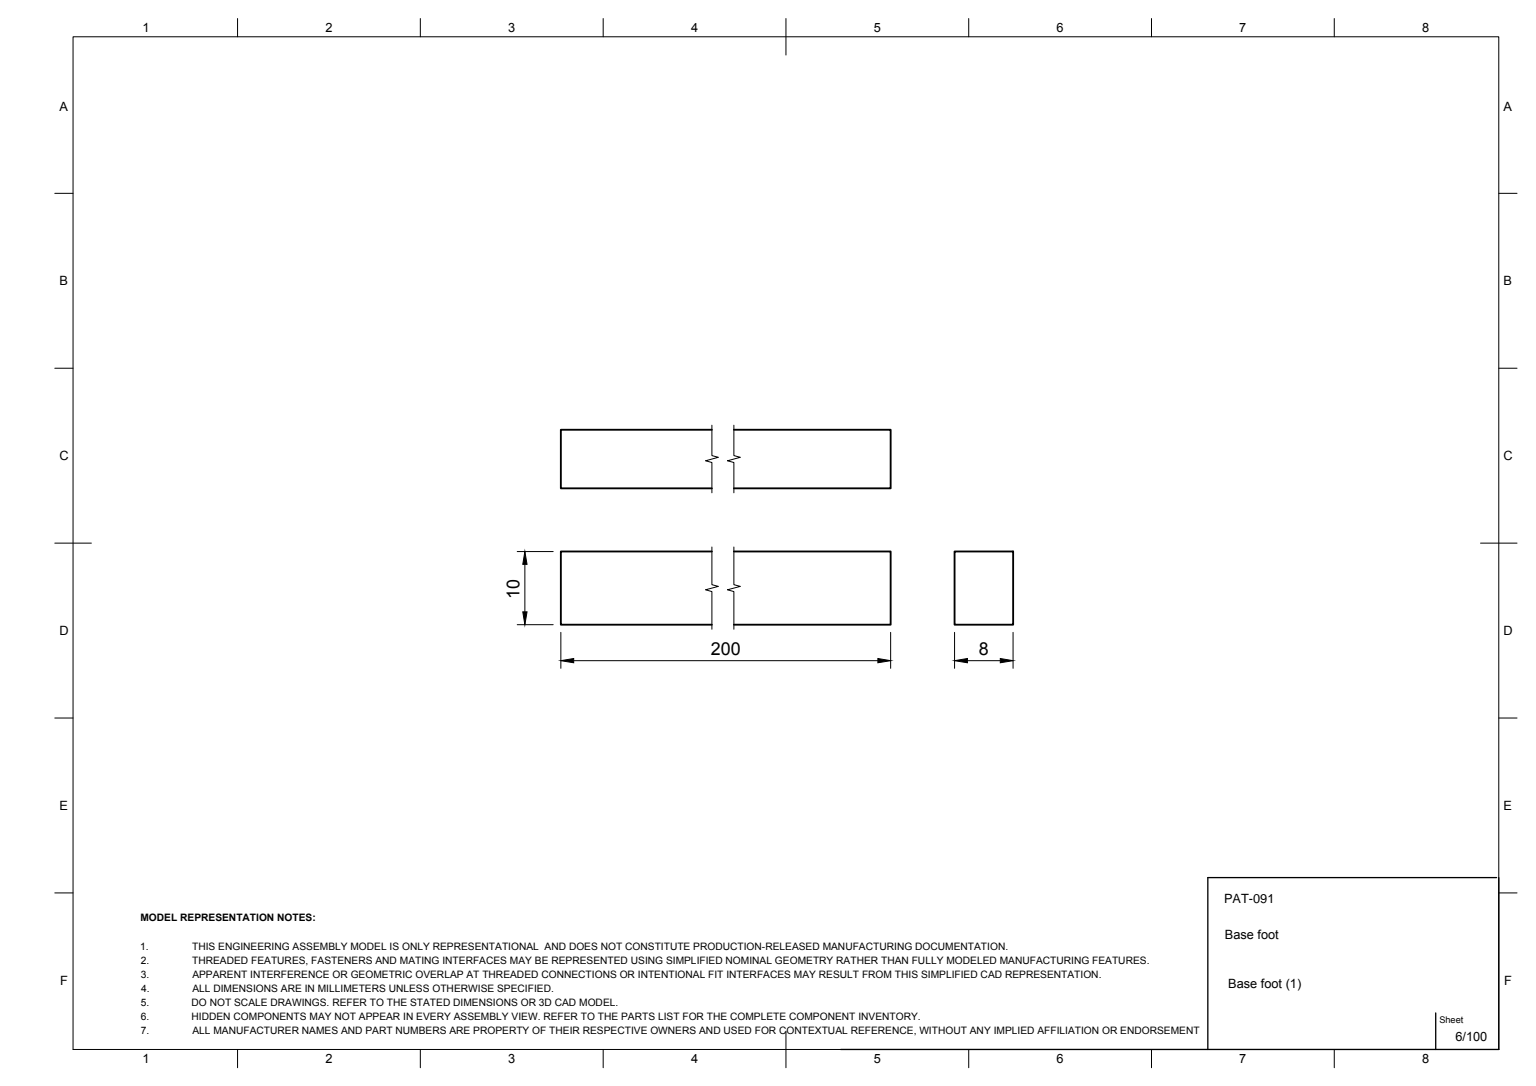
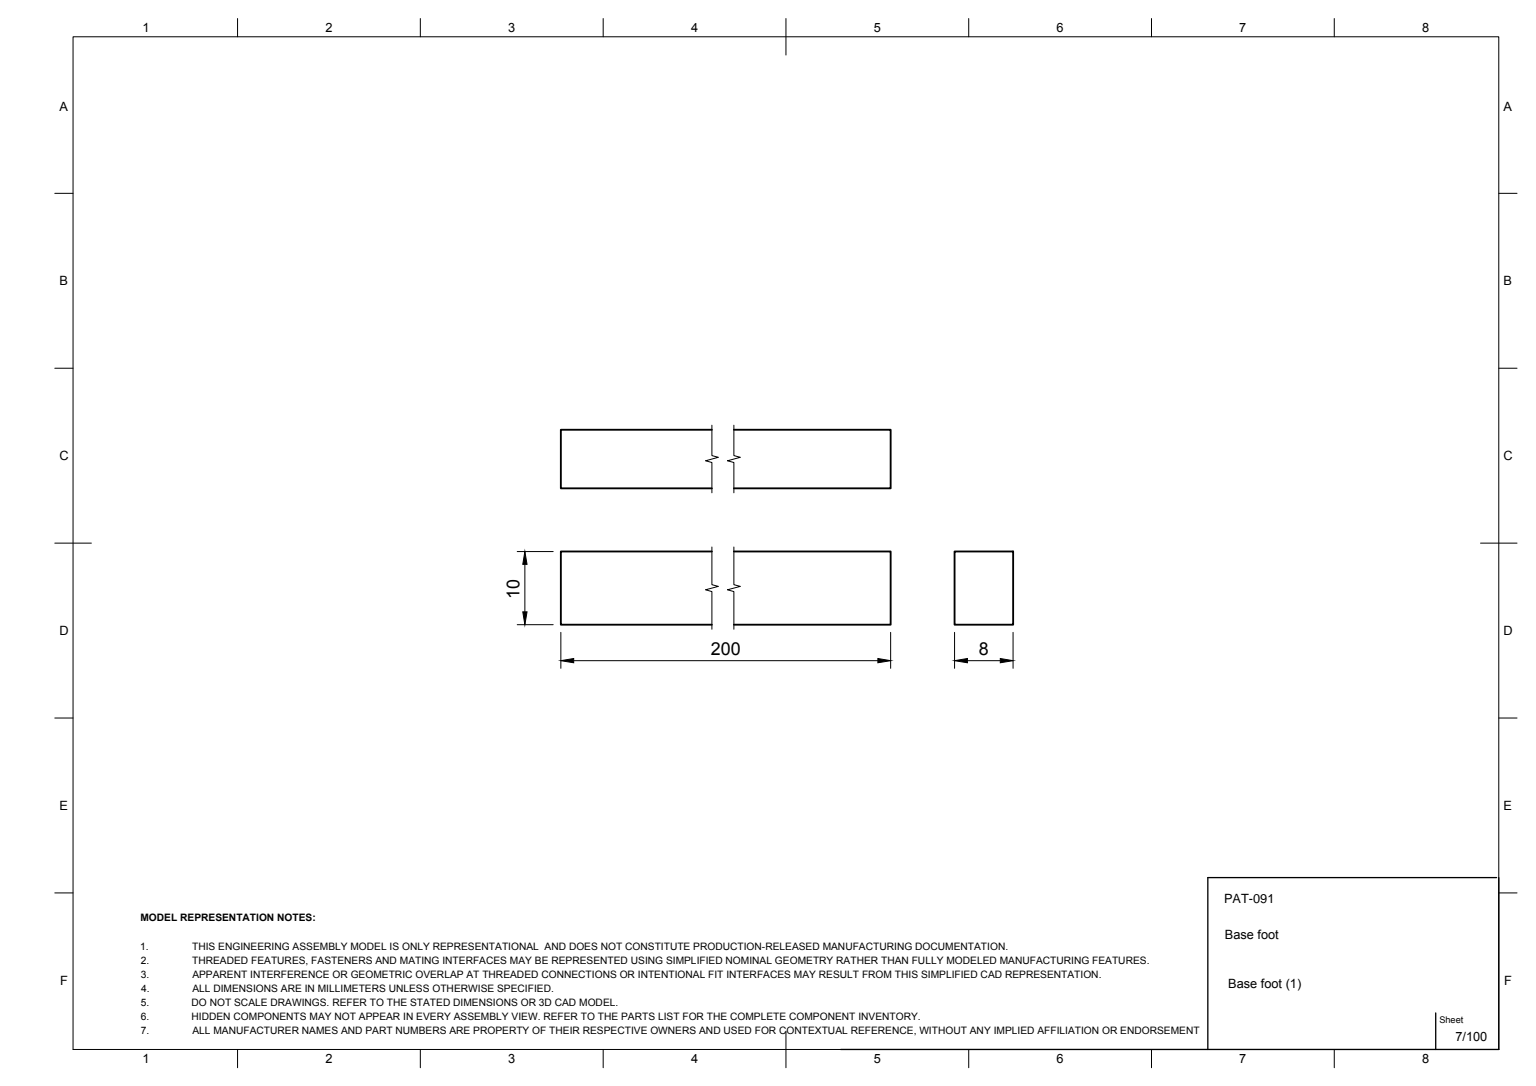
ISO-10303-21;
HEADER;
/* Generated by software containing ST-Developer
 * from STEP Tools, Inc. (www.steptools.com) 
 */

FILE_DESCRIPTION(
/* description */ ('PAT-091'),
/* implementation_level */ '2;1');

FILE_NAME(
/* name */ 'Base foot (1).step',
/* time_stamp */ '2026-10-27T15:34:44-07:00',
/* author */ (''),
/* organization */ (''),
/* preprocessor_version */ 'ST-DEVELOPER v20.2',
/* originating_system */ 'Autodesk Translation Framework v15.17.0.0',
/* authorisation */ '');

FILE_SCHEMA (('AUTOMOTIVE_DESIGN { 1 0 10303 214 3 1 1 }'));
ENDSEC;

DATA;
#10=MECHANICAL_DESIGN_GEOMETRIC_PRESENTATION_REPRESENTATION('',(#973),#25100);
#753=SHAPE_REPRESENTATION_RELATIONSHIP('SRR','None',#25514,#863);
#863=ADVANCED_BREP_SHAPE_REPRESENTATION('',(#1097),#24984);
#973=STYLED_ITEM('',(#26170),#1097);
#1097=MANIFOLD_SOLID_BREP('Body1',#13250);
#1652=PLANE('',#14626);
#1653=PLANE('',#14627);
#1654=PLANE('',#14628);
#1655=PLANE('',#14629);
#1656=PLANE('',#14630);
#1657=PLANE('',#14631);
#2083=FACE_OUTER_BOUND('',#2917,.T.);
#2084=FACE_OUTER_BOUND('',#2918,.T.);
#2085=FACE_OUTER_BOUND('',#2919,.T.);
#2086=FACE_OUTER_BOUND('',#2920,.T.);
#2087=FACE_OUTER_BOUND('',#2921,.T.);
#2088=FACE_OUTER_BOUND('',#2922,.T.);
#2917=EDGE_LOOP('',(#9068,#9069,#9070,#9071));
#2918=EDGE_LOOP('',(#9072,#9073,#9074,#9075));
#2919=EDGE_LOOP('',(#9076,#9077,#9078,#9079));
#2920=EDGE_LOOP('',(#9080,#9081,#9082,#9083));
#2921=EDGE_LOOP('',(#9084,#9085,#9086,#9087));
#2922=EDGE_LOOP('',(#9088,#9089,#9090,#9091));
#4156=LINE('',#21082,#4896);
#4157=LINE('',#21084,#4897);
#4158=LINE('',#21086,#4898);
#4159=LINE('',#21087,#4899);
#4160=LINE('',#21090,#4900);
#4161=LINE('',#21092,#4901);
#4162=LINE('',#21093,#4902);
#4163=LINE('',#21096,#4903);
#4164=LINE('',#21098,#4904);
#4165=LINE('',#21099,#4905);
#4166=LINE('',#21101,#4906);
#4167=LINE('',#21102,#4907);
#4896=VECTOR('',#16584,1.);
#4897=VECTOR('',#16585,1.);
#4898=VECTOR('',#16586,1.);
#4899=VECTOR('',#16587,1.);
#4900=VECTOR('',#16590,1.);
#4901=VECTOR('',#16591,1.);
#4902=VECTOR('',#16592,1.);
#4903=VECTOR('',#16595,1.);
#4904=VECTOR('',#16596,1.);
#4905=VECTOR('',#16597,1.);
#4906=VECTOR('',#16600,1.);
#4907=VECTOR('',#16601,1.);
#6415=VERTEX_POINT('',#21080);
#6416=VERTEX_POINT('',#21081);
#6417=VERTEX_POINT('',#21083);
#6418=VERTEX_POINT('',#21085);
#6419=VERTEX_POINT('',#21089);
#6420=VERTEX_POINT('',#21091);
#6421=VERTEX_POINT('',#21095);
#6422=VERTEX_POINT('',#21097);
#7469=EDGE_CURVE('',#6415,#6416,#4156,.T.);
#7470=EDGE_CURVE('',#6416,#6417,#4157,.T.);
#7471=EDGE_CURVE('',#6418,#6417,#4158,.T.);
#7472=EDGE_CURVE('',#6415,#6418,#4159,.T.);
#7473=EDGE_CURVE('',#6419,#6415,#4160,.T.);
#7474=EDGE_CURVE('',#6420,#6418,#4161,.T.);
#7475=EDGE_CURVE('',#6419,#6420,#4162,.T.);
#7476=EDGE_CURVE('',#6421,#6419,#4163,.T.);
#7477=EDGE_CURVE('',#6422,#6420,#4164,.T.);
#7478=EDGE_CURVE('',#6421,#6422,#4165,.T.);
#7479=EDGE_CURVE('',#6416,#6421,#4166,.T.);
#7480=EDGE_CURVE('',#6417,#6422,#4167,.T.);
#9068=ORIENTED_EDGE('',*,*,#7469,.T.);
#9069=ORIENTED_EDGE('',*,*,#7470,.T.);
#9070=ORIENTED_EDGE('',*,*,#7471,.F.);
#9071=ORIENTED_EDGE('',*,*,#7472,.F.);
#9072=ORIENTED_EDGE('',*,*,#7473,.T.);
#9073=ORIENTED_EDGE('',*,*,#7472,.T.);
#9074=ORIENTED_EDGE('',*,*,#7474,.F.);
#9075=ORIENTED_EDGE('',*,*,#7475,.F.);
#9076=ORIENTED_EDGE('',*,*,#7476,.T.);
#9077=ORIENTED_EDGE('',*,*,#7475,.T.);
#9078=ORIENTED_EDGE('',*,*,#7477,.F.);
#9079=ORIENTED_EDGE('',*,*,#7478,.F.);
#9080=ORIENTED_EDGE('',*,*,#7479,.T.);
#9081=ORIENTED_EDGE('',*,*,#7478,.T.);
#9082=ORIENTED_EDGE('',*,*,#7480,.F.);
#9083=ORIENTED_EDGE('',*,*,#7470,.F.);
#9084=ORIENTED_EDGE('',*,*,#7480,.T.);
#9085=ORIENTED_EDGE('',*,*,#7477,.T.);
#9086=ORIENTED_EDGE('',*,*,#7474,.T.);
#9087=ORIENTED_EDGE('',*,*,#7471,.T.);
#9088=ORIENTED_EDGE('',*,*,#7479,.F.);
#9089=ORIENTED_EDGE('',*,*,#7469,.F.);
#9090=ORIENTED_EDGE('',*,*,#7473,.F.);
#9091=ORIENTED_EDGE('',*,*,#7476,.F.);
#12450=ADVANCED_FACE('',(#2083),#1652,.T.);
#12451=ADVANCED_FACE('',(#2084),#1653,.T.);
#12452=ADVANCED_FACE('',(#2085),#1654,.T.);
#12453=ADVANCED_FACE('',(#2086),#1655,.T.);
#12454=ADVANCED_FACE('',(#2087),#1656,.T.);
#12455=ADVANCED_FACE('',(#2088),#1657,.F.);
#13250=CLOSED_SHELL('',(#12450,#12451,#12452,#12453,#12454,#12455));
#14625=AXIS2_PLACEMENT_3D('',#21078,#16580,#16581);
#14626=AXIS2_PLACEMENT_3D('',#21079,#16582,#16583);
#14627=AXIS2_PLACEMENT_3D('',#21088,#16588,#16589);
#14628=AXIS2_PLACEMENT_3D('',#21094,#16593,#16594);
#14629=AXIS2_PLACEMENT_3D('',#21100,#16598,#16599);
#14630=AXIS2_PLACEMENT_3D('',#21103,#16602,#16603);
#14631=AXIS2_PLACEMENT_3D('',#21104,#16604,#16605);
#16580=DIRECTION('axis',(0.,0.,1.));
#16581=DIRECTION('refdir',(1.,0.,0.));
#16582=DIRECTION('center_axis',(0.,1.,0.));
#16583=DIRECTION('ref_axis',(-1.,0.,0.));
#16584=DIRECTION('',(-1.,0.,0.));
#16585=DIRECTION('',(0.,0.,1.));
#16586=DIRECTION('',(-1.,0.,0.));
#16587=DIRECTION('',(0.,0.,1.));
#16588=DIRECTION('center_axis',(1.,0.,0.));
#16589=DIRECTION('ref_axis',(0.,1.,0.));
#16590=DIRECTION('',(0.,1.,0.));
#16591=DIRECTION('',(0.,1.,0.));
#16592=DIRECTION('',(0.,0.,1.));
#16593=DIRECTION('center_axis',(0.,-1.,0.));
#16594=DIRECTION('ref_axis',(1.,0.,0.));
#16595=DIRECTION('',(1.,0.,0.));
#16596=DIRECTION('',(1.,0.,0.));
#16597=DIRECTION('',(0.,0.,1.));
#16598=DIRECTION('center_axis',(-1.,0.,0.));
#16599=DIRECTION('ref_axis',(0.,-1.,0.));
#16600=DIRECTION('',(0.,-1.,0.));
#16601=DIRECTION('',(0.,-1.,0.));
#16602=DIRECTION('center_axis',(0.,0.,1.));
#16603=DIRECTION('ref_axis',(1.,0.,0.));
#16604=DIRECTION('center_axis',(0.,0.,1.));
#16605=DIRECTION('ref_axis',(1.,0.,0.));
#21078=CARTESIAN_POINT('',(0.,0.,0.));
#21079=CARTESIAN_POINT('Origin',(48.,10.,-0.8));
#21080=CARTESIAN_POINT('',(48.,10.,-1.8));
#21081=CARTESIAN_POINT('',(47.,10.,-1.8));
#21082=CARTESIAN_POINT('',(47.75,10.,-1.8));
#21083=CARTESIAN_POINT('',(47.,10.,0.));
#21084=CARTESIAN_POINT('',(47.,10.,-0.8));
#21085=CARTESIAN_POINT('',(48.,10.,0.));
#21086=CARTESIAN_POINT('',(48.,10.,0.));
#21087=CARTESIAN_POINT('',(48.,10.,-0.8));
#21088=CARTESIAN_POINT('Origin',(48.,-10.,-0.8));
#21089=CARTESIAN_POINT('',(48.,-10.,-1.8));
#21090=CARTESIAN_POINT('',(48.,-5.,-1.8));
#21091=CARTESIAN_POINT('',(48.,-10.,0.));
#21092=CARTESIAN_POINT('',(48.,-10.,0.));
#21093=CARTESIAN_POINT('',(48.,-10.,-0.8));
#21094=CARTESIAN_POINT('Origin',(47.,-10.,-0.8));
#21095=CARTESIAN_POINT('',(47.,-10.,-1.8));
#21096=CARTESIAN_POINT('',(47.25,-10.,-1.8));
#21097=CARTESIAN_POINT('',(47.,-10.,0.));
#21098=CARTESIAN_POINT('',(47.,-10.,0.));
#21099=CARTESIAN_POINT('',(47.,-10.,-0.8));
#21100=CARTESIAN_POINT('Origin',(47.,10.,-0.8));
#21101=CARTESIAN_POINT('',(47.,5.,-1.8));
#21102=CARTESIAN_POINT('',(47.,10.,0.));
#21103=CARTESIAN_POINT('Origin',(47.5,0.,0.));
#21104=CARTESIAN_POINT('Origin',(47.5,0.,-1.8));
#24863=UNCERTAINTY_MEASURE_WITH_UNIT(LENGTH_MEASURE(0.001),#25101,
'DISTANCE_ACCURACY_VALUE',
'Maximum model space distance between geometric entities at asserted c
onnectivities');
#24979=UNCERTAINTY_MEASURE_WITH_UNIT(LENGTH_MEASURE(0.001),#25101,
'DISTANCE_ACCURACY_VALUE',
'Maximum model space distance between geometric entities at asserted c
onnectivities');
#24984=(
GEOMETRIC_REPRESENTATION_CONTEXT(3)
GLOBAL_UNCERTAINTY_ASSIGNED_CONTEXT((#24863))
GLOBAL_UNIT_ASSIGNED_CONTEXT((#25101,#25103,#25104))
REPRESENTATION_CONTEXT('','3D')
);
#25100=(
GEOMETRIC_REPRESENTATION_CONTEXT(3)
GLOBAL_UNCERTAINTY_ASSIGNED_CONTEXT((#24979))
GLOBAL_UNIT_ASSIGNED_CONTEXT((#25101,#25103,#25104))
REPRESENTATION_CONTEXT('','3D')
);
#25101=(
LENGTH_UNIT()
NAMED_UNIT(*)
SI_UNIT(.CENTI.,.METRE.)
);
#25103=(
NAMED_UNIT(*)
PLANE_ANGLE_UNIT()
SI_UNIT($,.RADIAN.)
);
#25104=(
NAMED_UNIT(*)
SI_UNIT($,.STERADIAN.)
SOLID_ANGLE_UNIT()
);
#25109=SHAPE_DEFINITION_REPRESENTATION(#25229,#25514);
#25229=PRODUCT_DEFINITION_SHAPE('',$,#25635);
#25514=SHAPE_REPRESENTATION('',(#14625),#24984);
#25630=PRODUCT_DEFINITION_CONTEXT('part definition',#25992,'design');
#25635=PRODUCT_DEFINITION('Base foot (1)','Base foot (1)',#25755,#25630);
#25755=PRODUCT_DEFINITION_FORMATION('',$,#25998);
#25992=APPLICATION_CONTEXT(
'Core Data for Automotive Mechanical Design Process');
#25993=PRODUCT_CONTEXT('part definition',#25992,'mechanical');
#25998=PRODUCT('Base foot (1)','Base foot (1)','Base foot (1)',(#25993));
#26164=COLOUR_RGB('Dark Blue',0.08,0.2,0.34);
#26165=FILL_AREA_STYLE_COLOUR('',#26164);
#26166=FILL_AREA_STYLE('',(#26165));
#26167=SURFACE_STYLE_FILL_AREA(#26166);
#26168=SURFACE_SIDE_STYLE('',(#26167));
#26169=SURFACE_STYLE_USAGE(.BOTH.,#26168);
#26170=PRESENTATION_STYLE_ASSIGNMENT((#26169));
ENDSEC;
END-ISO-10303-21;
